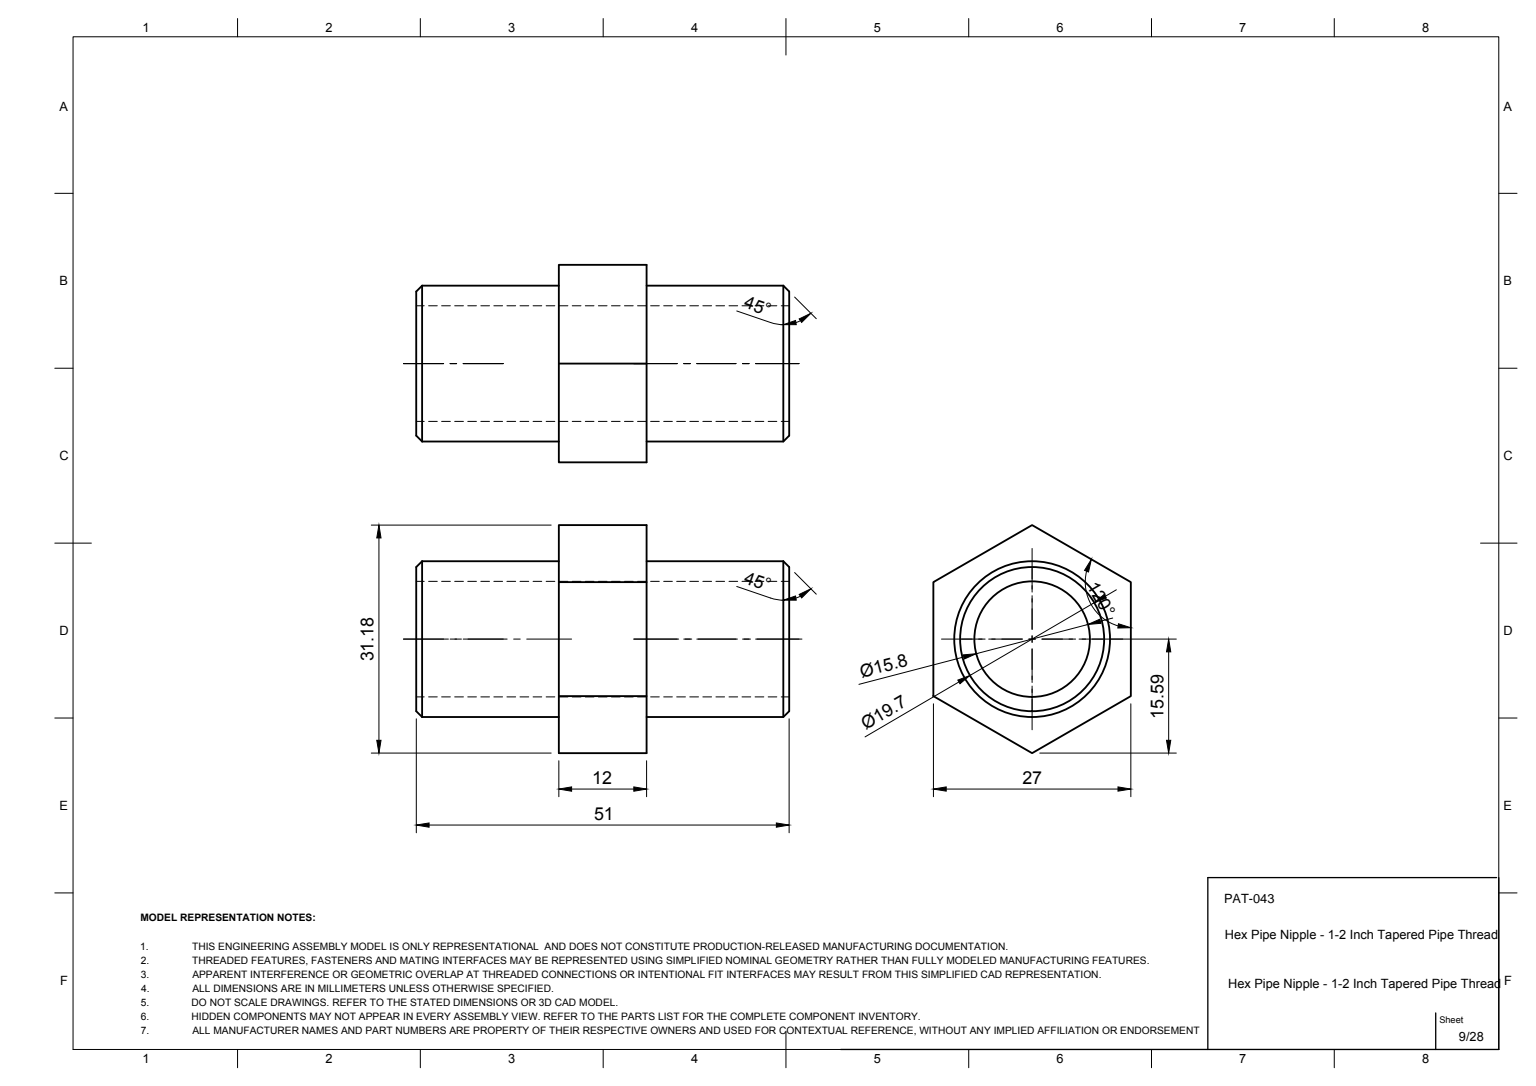
ISO-10303-21;
HEADER;
/* Generated by software containing ST-Developer
 * from STEP Tools, Inc. (www.steptools.com) 
 */

FILE_DESCRIPTION(
/* description */ ('Four-valve pipe header'),
/* implementation_level */ '2;1');

FILE_NAME(
/* name */ 'Hex Pipe Nipple - 1-2 Inch Tapered Pipe Thread.step',
/* time_stamp */ '2026-10-29T16:56:19-07:00',
/* author */ (''),
/* organization */ (''),
/* preprocessor_version */ 'ST-DEVELOPER v20.2',
/* originating_system */ 'Autodesk Translation Framework v15.17.0.0',
/* authorisation */ '');

FILE_SCHEMA (('AUTOMOTIVE_DESIGN { 1 0 10303 214 3 1 1 }'));
ENDSEC;

DATA;
#10=MECHANICAL_DESIGN_GEOMETRIC_PRESENTATION_REPRESENTATION('',(#349),#10119);
#272=CONICAL_SURFACE('',#6361,1.025,0.785398163397448);
#273=CONICAL_SURFACE('',#6364,1.025,0.785398163397448);
#297=SHAPE_REPRESENTATION_RELATIONSHIP('SRR','None',#10259,#323);
#323=ADVANCED_BREP_SHAPE_REPRESENTATION('',(#374),#10108);
#349=STYLED_ITEM('',(#10456),#374);
#374=MANIFOLD_SOLID_BREP('Body1',#5596);
#519=FACE_BOUND('',#1401,.T.);
#520=FACE_BOUND('',#1403,.T.);
#521=FACE_BOUND('',#1412,.T.);
#522=FACE_BOUND('',#1417,.T.);
#668=PLANE('',#6346);
#669=PLANE('',#6348);
#670=PLANE('',#6350);
#671=PLANE('',#6351);
#672=PLANE('',#6352);
#673=PLANE('',#6353);
#674=PLANE('',#6354);
#675=PLANE('',#6355);
#676=PLANE('',#6358);
#677=PLANE('',#6366);
#975=FACE_OUTER_BOUND('',#1400,.T.);
#976=FACE_OUTER_BOUND('',#1402,.T.);
#977=FACE_OUTER_BOUND('',#1404,.T.);
#978=FACE_OUTER_BOUND('',#1405,.T.);
#979=FACE_OUTER_BOUND('',#1406,.T.);
#980=FACE_OUTER_BOUND('',#1407,.T.);
#981=FACE_OUTER_BOUND('',#1408,.T.);
#982=FACE_OUTER_BOUND('',#1409,.T.);
#983=FACE_OUTER_BOUND('',#1410,.T.);
#984=FACE_OUTER_BOUND('',#1411,.T.);
#985=FACE_OUTER_BOUND('',#1413,.T.);
#986=FACE_OUTER_BOUND('',#1414,.T.);
#987=FACE_OUTER_BOUND('',#1415,.T.);
#988=FACE_OUTER_BOUND('',#1416,.T.);
#989=FACE_OUTER_BOUND('',#1418,.T.);
#1400=EDGE_LOOP('',(#4735,#4736,#4737,#4738,#4739,#4740));
#1401=EDGE_LOOP('',(#4741));
#1402=EDGE_LOOP('',(#4742,#4743,#4744,#4745,#4746,#4747));
#1403=EDGE_LOOP('',(#4748));
#1404=EDGE_LOOP('',(#4749,#4750,#4751,#4752));
#1405=EDGE_LOOP('',(#4753,#4754,#4755,#4756));
#1406=EDGE_LOOP('',(#4757,#4758,#4759,#4760));
#1407=EDGE_LOOP('',(#4761,#4762,#4763,#4764));
#1408=EDGE_LOOP('',(#4765,#4766,#4767,#4768));
#1409=EDGE_LOOP('',(#4769,#4770,#4771,#4772));
#1410=EDGE_LOOP('',(#4773,#4774,#4775,#4776));
#1411=EDGE_LOOP('',(#4777));
#1412=EDGE_LOOP('',(#4778));
#1413=EDGE_LOOP('',(#4779,#4780,#4781,#4782));
#1414=EDGE_LOOP('',(#4783,#4784,#4785,#4786));
#1415=EDGE_LOOP('',(#4787,#4788,#4789,#4790));
#1416=EDGE_LOOP('',(#4791));
#1417=EDGE_LOOP('',(#4792));
#1418=EDGE_LOOP('',(#4793,#4794,#4795,#4796));
#1784=LINE('',#9551,#2202);
#1785=LINE('',#9553,#2203);
#1786=LINE('',#9555,#2204);
#1787=LINE('',#9557,#2205);
#1788=LINE('',#9559,#2206);
#1789=LINE('',#9560,#2207);
#1790=LINE('',#9566,#2208);
#1791=LINE('',#9568,#2209);
#1792=LINE('',#9570,#2210);
#1793=LINE('',#9572,#2211);
#1794=LINE('',#9574,#2212);
#1795=LINE('',#9575,#2213);
#1796=LINE('',#9579,#2214);
#1797=LINE('',#9580,#2215);
#1798=LINE('',#9582,#2216);
#1799=LINE('',#9584,#2217);
#1800=LINE('',#9586,#2218);
#1801=LINE('',#9588,#2219);
#1802=LINE('',#9592,#2220);
#1803=LINE('',#9600,#2221);
#1804=LINE('',#9604,#2222);
#1805=LINE('',#9608,#2223);
#1806=LINE('',#9613,#2224);
#2202=VECTOR('',#7737,1.);
#2203=VECTOR('',#7738,1.);
#2204=VECTOR('',#7739,1.);
#2205=VECTOR('',#7740,1.);
#2206=VECTOR('',#7741,1.);
#2207=VECTOR('',#7742,1.);
#2208=VECTOR('',#7747,1.);
#2209=VECTOR('',#7748,1.);
#2210=VECTOR('',#7749,1.);
#2211=VECTOR('',#7750,1.);
#2212=VECTOR('',#7751,1.);
#2213=VECTOR('',#7752,1.);
#2214=VECTOR('',#7757,1.);
#2215=VECTOR('',#7758,1.);
#2216=VECTOR('',#7761,1.);
#2217=VECTOR('',#7764,1.);
#2218=VECTOR('',#7767,1.);
#2219=VECTOR('',#7770,1.);
#2220=VECTOR('',#7775,1.065);
#2221=VECTOR('',#7786,1.025);
#2222=VECTOR('',#7791,1.065);
#2223=VECTOR('',#7796,1.025);
#2224=VECTOR('',#7803,0.79);
#2527=CIRCLE('',#6347,1.065);
#2528=CIRCLE('',#6349,1.065);
#2529=CIRCLE('',#6357,1.065);
#2530=CIRCLE('',#6359,0.985);
#2531=CIRCLE('',#6360,0.79);
#2532=CIRCLE('',#6363,1.065);
#2533=CIRCLE('',#6365,0.985);
#2534=CIRCLE('',#6367,0.79);
#2904=VERTEX_POINT('',#9549);
#2905=VERTEX_POINT('',#9550);
#2906=VERTEX_POINT('',#9552);
#2907=VERTEX_POINT('',#9554);
#2908=VERTEX_POINT('',#9556);
#2909=VERTEX_POINT('',#9558);
#2910=VERTEX_POINT('',#9561);
#2911=VERTEX_POINT('',#9564);
#2912=VERTEX_POINT('',#9565);
#2913=VERTEX_POINT('',#9567);
#2914=VERTEX_POINT('',#9569);
#2915=VERTEX_POINT('',#9571);
#2916=VERTEX_POINT('',#9573);
#2917=VERTEX_POINT('',#9576);
#2918=VERTEX_POINT('',#9591);
#2919=VERTEX_POINT('',#9595);
#2920=VERTEX_POINT('',#9597);
#2921=VERTEX_POINT('',#9602);
#2922=VERTEX_POINT('',#9606);
#2923=VERTEX_POINT('',#9610);
#3534=EDGE_CURVE('',#2904,#2905,#1784,.T.);
#3535=EDGE_CURVE('',#2905,#2906,#1785,.T.);
#3536=EDGE_CURVE('',#2906,#2907,#1786,.T.);
#3537=EDGE_CURVE('',#2907,#2908,#1787,.T.);
#3538=EDGE_CURVE('',#2908,#2909,#1788,.T.);
#3539=EDGE_CURVE('',#2909,#2904,#1789,.T.);
#3540=EDGE_CURVE('',#2910,#2910,#2527,.T.);
#3541=EDGE_CURVE('',#2911,#2912,#1790,.T.);
#3542=EDGE_CURVE('',#2912,#2913,#1791,.T.);
#3543=EDGE_CURVE('',#2913,#2914,#1792,.T.);
#3544=EDGE_CURVE('',#2914,#2915,#1793,.T.);
#3545=EDGE_CURVE('',#2915,#2916,#1794,.T.);
#3546=EDGE_CURVE('',#2916,#2911,#1795,.T.);
#3547=EDGE_CURVE('',#2917,#2917,#2528,.T.);
#3548=EDGE_CURVE('',#2911,#2905,#1796,.T.);
#3549=EDGE_CURVE('',#2906,#2916,#1797,.T.);
#3550=EDGE_CURVE('',#2907,#2915,#1798,.T.);
#3551=EDGE_CURVE('',#2908,#2914,#1799,.T.);
#3552=EDGE_CURVE('',#2909,#2913,#1800,.T.);
#3553=EDGE_CURVE('',#2904,#2912,#1801,.T.);
#3554=EDGE_CURVE('',#2917,#2918,#1802,.T.);
#3555=EDGE_CURVE('',#2918,#2918,#2529,.T.);
#3556=EDGE_CURVE('',#2919,#2919,#2530,.T.);
#3557=EDGE_CURVE('',#2920,#2920,#2531,.T.);
#3558=EDGE_CURVE('',#2918,#2919,#1803,.T.);
#3559=EDGE_CURVE('',#2921,#2921,#2532,.T.);
#3560=EDGE_CURVE('',#2921,#2910,#1804,.T.);
#3561=EDGE_CURVE('',#2922,#2922,#2533,.T.);
#3562=EDGE_CURVE('',#2922,#2921,#1805,.T.);
#3563=EDGE_CURVE('',#2923,#2923,#2534,.T.);
#3564=EDGE_CURVE('',#2923,#2920,#1806,.T.);
#4735=ORIENTED_EDGE('',*,*,#3534,.T.);
#4736=ORIENTED_EDGE('',*,*,#3535,.T.);
#4737=ORIENTED_EDGE('',*,*,#3536,.T.);
#4738=ORIENTED_EDGE('',*,*,#3537,.T.);
#4739=ORIENTED_EDGE('',*,*,#3538,.T.);
#4740=ORIENTED_EDGE('',*,*,#3539,.T.);
#4741=ORIENTED_EDGE('',*,*,#3540,.F.);
#4742=ORIENTED_EDGE('',*,*,#3541,.T.);
#4743=ORIENTED_EDGE('',*,*,#3542,.T.);
#4744=ORIENTED_EDGE('',*,*,#3543,.T.);
#4745=ORIENTED_EDGE('',*,*,#3544,.T.);
#4746=ORIENTED_EDGE('',*,*,#3545,.T.);
#4747=ORIENTED_EDGE('',*,*,#3546,.T.);
#4748=ORIENTED_EDGE('',*,*,#3547,.F.);
#4749=ORIENTED_EDGE('',*,*,#3548,.F.);
#4750=ORIENTED_EDGE('',*,*,#3546,.F.);
#4751=ORIENTED_EDGE('',*,*,#3549,.F.);
#4752=ORIENTED_EDGE('',*,*,#3535,.F.);
#4753=ORIENTED_EDGE('',*,*,#3549,.T.);
#4754=ORIENTED_EDGE('',*,*,#3545,.F.);
#4755=ORIENTED_EDGE('',*,*,#3550,.F.);
#4756=ORIENTED_EDGE('',*,*,#3536,.F.);
#4757=ORIENTED_EDGE('',*,*,#3550,.T.);
#4758=ORIENTED_EDGE('',*,*,#3544,.F.);
#4759=ORIENTED_EDGE('',*,*,#3551,.F.);
#4760=ORIENTED_EDGE('',*,*,#3537,.F.);
#4761=ORIENTED_EDGE('',*,*,#3551,.T.);
#4762=ORIENTED_EDGE('',*,*,#3543,.F.);
#4763=ORIENTED_EDGE('',*,*,#3552,.F.);
#4764=ORIENTED_EDGE('',*,*,#3538,.F.);
#4765=ORIENTED_EDGE('',*,*,#3552,.T.);
#4766=ORIENTED_EDGE('',*,*,#3542,.F.);
#4767=ORIENTED_EDGE('',*,*,#3553,.F.);
#4768=ORIENTED_EDGE('',*,*,#3539,.F.);
#4769=ORIENTED_EDGE('',*,*,#3553,.T.);
#4770=ORIENTED_EDGE('',*,*,#3541,.F.);
#4771=ORIENTED_EDGE('',*,*,#3548,.T.);
#4772=ORIENTED_EDGE('',*,*,#3534,.F.);
#4773=ORIENTED_EDGE('',*,*,#3547,.T.);
#4774=ORIENTED_EDGE('',*,*,#3554,.T.);
#4775=ORIENTED_EDGE('',*,*,#3555,.T.);
#4776=ORIENTED_EDGE('',*,*,#3554,.F.);
#4777=ORIENTED_EDGE('',*,*,#3556,.F.);
#4778=ORIENTED_EDGE('',*,*,#3557,.T.);
#4779=ORIENTED_EDGE('',*,*,#3555,.F.);
#4780=ORIENTED_EDGE('',*,*,#3558,.T.);
#4781=ORIENTED_EDGE('',*,*,#3556,.T.);
#4782=ORIENTED_EDGE('',*,*,#3558,.F.);
#4783=ORIENTED_EDGE('',*,*,#3559,.F.);
#4784=ORIENTED_EDGE('',*,*,#3560,.T.);
#4785=ORIENTED_EDGE('',*,*,#3540,.T.);
#4786=ORIENTED_EDGE('',*,*,#3560,.F.);
#4787=ORIENTED_EDGE('',*,*,#3561,.F.);
#4788=ORIENTED_EDGE('',*,*,#3562,.T.);
#4789=ORIENTED_EDGE('',*,*,#3559,.T.);
#4790=ORIENTED_EDGE('',*,*,#3562,.F.);
#4791=ORIENTED_EDGE('',*,*,#3561,.T.);
#4792=ORIENTED_EDGE('',*,*,#3563,.F.);
#4793=ORIENTED_EDGE('',*,*,#3563,.T.);
#4794=ORIENTED_EDGE('',*,*,#3564,.T.);
#4795=ORIENTED_EDGE('',*,*,#3557,.F.);
#4796=ORIENTED_EDGE('',*,*,#3564,.F.);
#5232=CYLINDRICAL_SURFACE('',#6356,1.065);
#5233=CYLINDRICAL_SURFACE('',#6362,1.065);
#5234=CYLINDRICAL_SURFACE('',#6368,0.79);
#5475=ADVANCED_FACE('',(#975,#519),#668,.F.);
#5476=ADVANCED_FACE('',(#976,#520),#669,.T.);
#5477=ADVANCED_FACE('',(#977),#670,.T.);
#5478=ADVANCED_FACE('',(#978),#671,.T.);
#5479=ADVANCED_FACE('',(#979),#672,.T.);
#5480=ADVANCED_FACE('',(#980),#673,.T.);
#5481=ADVANCED_FACE('',(#981),#674,.T.);
#5482=ADVANCED_FACE('',(#982),#675,.T.);
#5483=ADVANCED_FACE('',(#983),#5232,.T.);
#5484=ADVANCED_FACE('',(#984,#521),#676,.T.);
#5485=ADVANCED_FACE('',(#985),#272,.T.);
#5486=ADVANCED_FACE('',(#986),#5233,.T.);
#5487=ADVANCED_FACE('',(#987),#273,.T.);
#5488=ADVANCED_FACE('',(#988,#522),#677,.T.);
#5489=ADVANCED_FACE('',(#989),#5234,.F.);
#5596=CLOSED_SHELL('',(#5475,#5476,#5477,#5478,#5479,#5480,#5481,#5482,
#5483,#5484,#5485,#5486,#5487,#5488,#5489));
#6345=AXIS2_PLACEMENT_3D('',#9547,#7733,#7734);
#6346=AXIS2_PLACEMENT_3D('',#9548,#7735,#7736);
#6347=AXIS2_PLACEMENT_3D('',#9562,#7743,#7744);
#6348=AXIS2_PLACEMENT_3D('',#9563,#7745,#7746);
#6349=AXIS2_PLACEMENT_3D('',#9577,#7753,#7754);
#6350=AXIS2_PLACEMENT_3D('',#9578,#7755,#7756);
#6351=AXIS2_PLACEMENT_3D('',#9581,#7759,#7760);
#6352=AXIS2_PLACEMENT_3D('',#9583,#7762,#7763);
#6353=AXIS2_PLACEMENT_3D('',#9585,#7765,#7766);
#6354=AXIS2_PLACEMENT_3D('',#9587,#7768,#7769);
#6355=AXIS2_PLACEMENT_3D('',#9589,#7771,#7772);
#6356=AXIS2_PLACEMENT_3D('',#9590,#7773,#7774);
#6357=AXIS2_PLACEMENT_3D('',#9593,#7776,#7777);
#6358=AXIS2_PLACEMENT_3D('',#9594,#7778,#7779);
#6359=AXIS2_PLACEMENT_3D('',#9596,#7780,#7781);
#6360=AXIS2_PLACEMENT_3D('',#9598,#7782,#7783);
#6361=AXIS2_PLACEMENT_3D('',#9599,#7784,#7785);
#6362=AXIS2_PLACEMENT_3D('',#9601,#7787,#7788);
#6363=AXIS2_PLACEMENT_3D('',#9603,#7789,#7790);
#6364=AXIS2_PLACEMENT_3D('',#9605,#7792,#7793);
#6365=AXIS2_PLACEMENT_3D('',#9607,#7794,#7795);
#6366=AXIS2_PLACEMENT_3D('',#9609,#7797,#7798);
#6367=AXIS2_PLACEMENT_3D('',#9611,#7799,#7800);
#6368=AXIS2_PLACEMENT_3D('',#9612,#7801,#7802);
#7733=DIRECTION('axis',(0.,0.,1.));
#7734=DIRECTION('refdir',(1.,0.,0.));
#7735=DIRECTION('center_axis',(0.,1.,0.));
#7736=DIRECTION('ref_axis',(1.,0.,0.));
#7737=DIRECTION('',(-0.5,0.,0.866025403784439));
#7738=DIRECTION('',(-1.,0.,-2.84883360945713E-16));
#7739=DIRECTION('',(-0.5,0.,-0.866025403784439));
#7740=DIRECTION('',(0.5,0.,-0.866025403784439));
#7741=DIRECTION('',(1.,0.,0.));
#7742=DIRECTION('',(0.5,0.,0.866025403784439));
#7743=DIRECTION('center_axis',(0.,-1.,0.));
#7744=DIRECTION('ref_axis',(1.,0.,0.));
#7745=DIRECTION('center_axis',(0.,1.,0.));
#7746=DIRECTION('ref_axis',(1.,0.,0.));
#7747=DIRECTION('',(0.5,0.,-0.866025403784439));
#7748=DIRECTION('',(-0.5,0.,-0.866025403784439));
#7749=DIRECTION('',(-1.,0.,0.));
#7750=DIRECTION('',(-0.5,0.,0.866025403784439));
#7751=DIRECTION('',(0.5,0.,0.866025403784439));
#7752=DIRECTION('',(1.,0.,2.84883360945713E-16));
#7753=DIRECTION('center_axis',(0.,1.,0.));
#7754=DIRECTION('ref_axis',(1.,0.,0.));
#7755=DIRECTION('center_axis',(-2.84883360945713E-16,0.,1.));
#7756=DIRECTION('ref_axis',(1.,0.,2.84883360945713E-16));
#7757=DIRECTION('',(0.,-1.,0.));
#7758=DIRECTION('',(0.,1.,0.));
#7759=DIRECTION('center_axis',(-0.866025403784439,0.,0.5));
#7760=DIRECTION('ref_axis',(0.5,0.,0.866025403784439));
#7761=DIRECTION('',(0.,1.,0.));
#7762=DIRECTION('center_axis',(-0.866025403784439,0.,-0.5));
#7763=DIRECTION('ref_axis',(-0.5,0.,0.866025403784439));
#7764=DIRECTION('',(0.,1.,0.));
#7765=DIRECTION('center_axis',(0.,0.,-1.));
#7766=DIRECTION('ref_axis',(-1.,0.,0.));
#7767=DIRECTION('',(0.,1.,0.));
#7768=DIRECTION('center_axis',(0.866025403784439,0.,-0.5));
#7769=DIRECTION('ref_axis',(-0.5,0.,-0.866025403784439));
#7770=DIRECTION('',(0.,1.,0.));
#7771=DIRECTION('center_axis',(0.866025403784439,0.,0.5));
#7772=DIRECTION('ref_axis',(0.5,0.,-0.866025403784439));
#7773=DIRECTION('center_axis',(0.,-1.,0.));
#7774=DIRECTION('ref_axis',(1.,0.,0.));
#7775=DIRECTION('',(0.,1.,0.));
#7776=DIRECTION('center_axis',(0.,-1.,0.));
#7777=DIRECTION('ref_axis',(1.,0.,0.));
#7778=DIRECTION('center_axis',(0.,1.,0.));
#7779=DIRECTION('ref_axis',(0.,0.,1.));
#7780=DIRECTION('center_axis',(0.,-1.,0.));
#7781=DIRECTION('ref_axis',(1.,0.,0.));
#7782=DIRECTION('center_axis',(0.,-1.,0.));
#7783=DIRECTION('ref_axis',(1.,0.,0.));
#7784=DIRECTION('center_axis',(0.,-1.,0.));
#7785=DIRECTION('ref_axis',(1.,0.,0.));
#7786=DIRECTION('',(0.707106781186547,0.707106781186548,8.65956056235493E-17));
#7787=DIRECTION('center_axis',(0.,-1.,0.));
#7788=DIRECTION('ref_axis',(1.,0.,0.));
#7789=DIRECTION('center_axis',(0.,-1.,0.));
#7790=DIRECTION('ref_axis',(1.,0.,0.));
#7791=DIRECTION('',(0.,1.,0.));
#7792=DIRECTION('center_axis',(0.,1.,0.));
#7793=DIRECTION('ref_axis',(1.,0.,0.));
#7794=DIRECTION('center_axis',(0.,-1.,0.));
#7795=DIRECTION('ref_axis',(1.,0.,0.));
#7796=DIRECTION('',(-0.707106781186547,0.707106781186548,-8.65956056235493E-17));
#7797=DIRECTION('center_axis',(0.,-1.,0.));
#7798=DIRECTION('ref_axis',(0.,0.,-1.));
#7799=DIRECTION('center_axis',(0.,-1.,0.));
#7800=DIRECTION('ref_axis',(1.,0.,0.));
#7801=DIRECTION('center_axis',(0.,-1.,0.));
#7802=DIRECTION('ref_axis',(1.,0.,0.));
#7803=DIRECTION('',(0.,1.,0.));
#9547=CARTESIAN_POINT('',(0.,0.,0.));
#9548=CARTESIAN_POINT('Origin',(0.,-0.6,0.));
#9549=CARTESIAN_POINT('',(1.55884572681199,-0.6,0.));
#9550=CARTESIAN_POINT('',(0.779422863405995,-0.6,1.35));
#9551=CARTESIAN_POINT('',(0.779422863405995,-0.6,1.35));
#9552=CARTESIAN_POINT('',(-0.779422863405996,-0.6,1.35));
#9553=CARTESIAN_POINT('',(-0.779422863405996,-0.6,1.35));
#9554=CARTESIAN_POINT('',(-1.55884572681199,-0.6,-1.90903542970483E-16));
#9555=CARTESIAN_POINT('',(-1.55884572681199,-0.6,-1.90903542970483E-16));
#9556=CARTESIAN_POINT('',(-0.779422863405995,-0.6,-1.35));
#9557=CARTESIAN_POINT('',(-0.779422863405995,-0.6,-1.35));
#9558=CARTESIAN_POINT('',(0.779422863405995,-0.6,-1.35));
#9559=CARTESIAN_POINT('',(0.779422863405995,-0.6,-1.35));
#9560=CARTESIAN_POINT('',(1.55884572681199,-0.6,0.));
#9561=CARTESIAN_POINT('',(-1.065,-0.6,-1.30424884109193E-16));
#9562=CARTESIAN_POINT('Origin',(0.,-0.6,0.));
#9563=CARTESIAN_POINT('Origin',(0.,0.6,0.));
#9564=CARTESIAN_POINT('',(0.779422863405995,0.6,1.35));
#9565=CARTESIAN_POINT('',(1.55884572681199,0.6,0.));
#9566=CARTESIAN_POINT('',(0.779422863405995,0.6,1.35));
#9567=CARTESIAN_POINT('',(0.779422863405995,0.6,-1.35));
#9568=CARTESIAN_POINT('',(1.55884572681199,0.6,0.));
#9569=CARTESIAN_POINT('',(-0.779422863405995,0.6,-1.35));
#9570=CARTESIAN_POINT('',(0.779422863405995,0.6,-1.35));
#9571=CARTESIAN_POINT('',(-1.55884572681199,0.6,-1.90903542970483E-16));
#9572=CARTESIAN_POINT('',(-0.779422863405995,0.6,-1.35));
#9573=CARTESIAN_POINT('',(-0.779422863405996,0.6,1.35));
#9574=CARTESIAN_POINT('',(-1.55884572681199,0.6,-1.90903542970483E-16));
#9575=CARTESIAN_POINT('',(-0.779422863405996,0.6,1.35));
#9576=CARTESIAN_POINT('',(-1.065,0.6,1.30424884109193E-16));
#9577=CARTESIAN_POINT('Origin',(0.,0.6,0.));
#9578=CARTESIAN_POINT('Origin',(-0.779422863405996,0.,1.35));
#9579=CARTESIAN_POINT('',(0.779422863405995,0.,1.35));
#9580=CARTESIAN_POINT('',(-0.779422863405996,0.,1.35));
#9581=CARTESIAN_POINT('Origin',(-1.55884572681199,0.,-1.90903542970483E-16));
#9582=CARTESIAN_POINT('',(-1.55884572681199,0.,-1.90903542970483E-16));
#9583=CARTESIAN_POINT('Origin',(-0.779422863405995,0.,-1.35));
#9584=CARTESIAN_POINT('',(-0.779422863405995,0.,-1.35));
#9585=CARTESIAN_POINT('Origin',(0.779422863405995,0.,-1.35));
#9586=CARTESIAN_POINT('',(0.779422863405995,0.,-1.35));
#9587=CARTESIAN_POINT('Origin',(1.55884572681199,0.,0.));
#9588=CARTESIAN_POINT('',(1.55884572681199,0.,0.));
#9589=CARTESIAN_POINT('Origin',(0.779422863405995,0.,1.35));
#9590=CARTESIAN_POINT('Origin',(0.,0.,0.));
#9591=CARTESIAN_POINT('',(-1.065,2.47,-1.30424884109193E-16));
#9592=CARTESIAN_POINT('',(-1.065,0.,-1.30424884109193E-16));
#9593=CARTESIAN_POINT('Origin',(0.,2.47,0.));
#9594=CARTESIAN_POINT('Origin',(0.985,2.55,0.));
#9595=CARTESIAN_POINT('',(-0.985,2.55,-1.20627709716014E-16));
#9596=CARTESIAN_POINT('Origin',(0.,2.55,0.));
#9597=CARTESIAN_POINT('',(-0.79,2.55,-9.67470971326409E-17));
#9598=CARTESIAN_POINT('Origin',(0.,2.55,0.));
#9599=CARTESIAN_POINT('Origin',(0.,2.51,0.));
#9600=CARTESIAN_POINT('',(-1.025,2.51,-1.25526296912604E-16));
#9601=CARTESIAN_POINT('Origin',(0.,0.,0.));
#9602=CARTESIAN_POINT('',(-1.065,-2.47,-1.30424884109193E-16));
#9603=CARTESIAN_POINT('Origin',(0.,-2.47,0.));
#9604=CARTESIAN_POINT('',(-1.065,0.,-1.30424884109193E-16));
#9605=CARTESIAN_POINT('Origin',(0.,-2.51,0.));
#9606=CARTESIAN_POINT('',(-0.985,-2.55,-1.20627709716014E-16));
#9607=CARTESIAN_POINT('Origin',(0.,-2.55,0.));
#9608=CARTESIAN_POINT('',(-1.025,-2.51,-1.25526296912604E-16));
#9609=CARTESIAN_POINT('Origin',(0.79,-2.55,0.));
#9610=CARTESIAN_POINT('',(-0.79,-2.55,-9.67470971326409E-17));
#9611=CARTESIAN_POINT('Origin',(0.,-2.55,0.));
#9612=CARTESIAN_POINT('Origin',(0.,0.,0.));
#9613=CARTESIAN_POINT('',(-0.79,0.,-9.67470971326409E-17));
#10077=UNCERTAINTY_MEASURE_WITH_UNIT(LENGTH_MEASURE(0.001),#10120,
'DISTANCE_ACCURACY_VALUE',
'Maximum model space distance between geometric entities at asserted c
onnectivities');
#10088=UNCERTAINTY_MEASURE_WITH_UNIT(LENGTH_MEASURE(0.001),#10120,
'DISTANCE_ACCURACY_VALUE',
'Maximum model space distance between geometric entities at asserted c
onnectivities');
#10108=(
GEOMETRIC_REPRESENTATION_CONTEXT(3)
GLOBAL_UNCERTAINTY_ASSIGNED_CONTEXT((#10077))
GLOBAL_UNIT_ASSIGNED_CONTEXT((#10120,#10122,#10123))
REPRESENTATION_CONTEXT('','3D')
);
#10119=(
GEOMETRIC_REPRESENTATION_CONTEXT(3)
GLOBAL_UNCERTAINTY_ASSIGNED_CONTEXT((#10088))
GLOBAL_UNIT_ASSIGNED_CONTEXT((#10120,#10122,#10123))
REPRESENTATION_CONTEXT('','3D')
);
#10120=(
LENGTH_UNIT()
NAMED_UNIT(*)
SI_UNIT(.CENTI.,.METRE.)
);
#10122=(
NAMED_UNIT(*)
PLANE_ANGLE_UNIT()
SI_UNIT($,.RADIAN.)
);
#10123=(
NAMED_UNIT(*)
SI_UNIT($,.STERADIAN.)
SOLID_ANGLE_UNIT()
);
#10143=SHAPE_DEFINITION_REPRESENTATION(#10173,#10259);
#10173=PRODUCT_DEFINITION_SHAPE('',$,#10290);
#10259=SHAPE_REPRESENTATION('',(#6345),#10108);
#10270=PRODUCT_DEFINITION_CONTEXT('part definition',#10362,'design');
#10290=PRODUCT_DEFINITION(
'Hex Pipe Nipple - 1-2 Inch Tapered Pipe Thread',
'Hex Pipe Nipple - 1-2 Inch Tapered Pipe Thread',#10320,#10270);
#10320=PRODUCT_DEFINITION_FORMATION('',$,#10383);
#10362=APPLICATION_CONTEXT(
'Core Data for Automotive Mechanical Design Process');
#10363=PRODUCT_CONTEXT('part definition',#10362,'mechanical');
#10383=PRODUCT('Hex Pipe Nipple - 1-2 Inch Tapered Pipe Thread',
'Hex Pipe Nipple - 1-2 Inch Tapered Pipe Thread',
'Hex Pipe Nipple - 1-2 Inch Tapered Pipe Thread',(#10363));
#10450=COLOUR_RGB('Light Blue',0.38,0.62,0.78);
#10451=FILL_AREA_STYLE_COLOUR('',#10450);
#10452=FILL_AREA_STYLE('',(#10451));
#10453=SURFACE_STYLE_FILL_AREA(#10452);
#10454=SURFACE_SIDE_STYLE('',(#10453));
#10455=SURFACE_STYLE_USAGE(.BOTH.,#10454);
#10456=PRESENTATION_STYLE_ASSIGNMENT((#10455));
ENDSEC;
END-ISO-10303-21;
